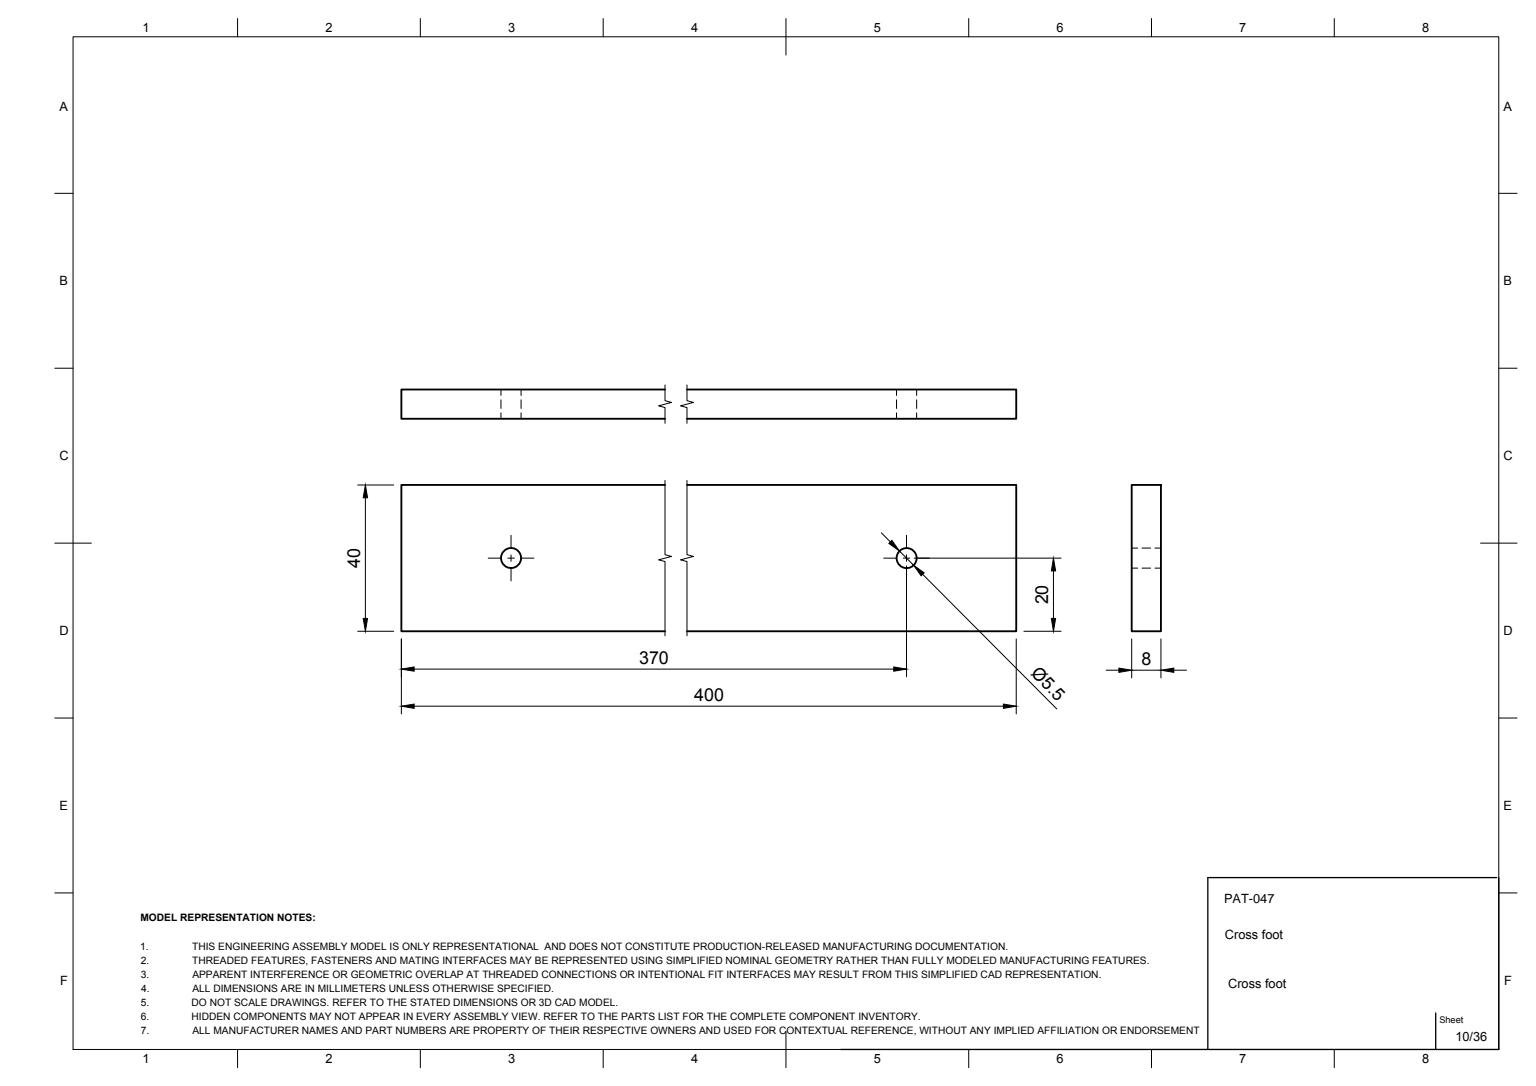
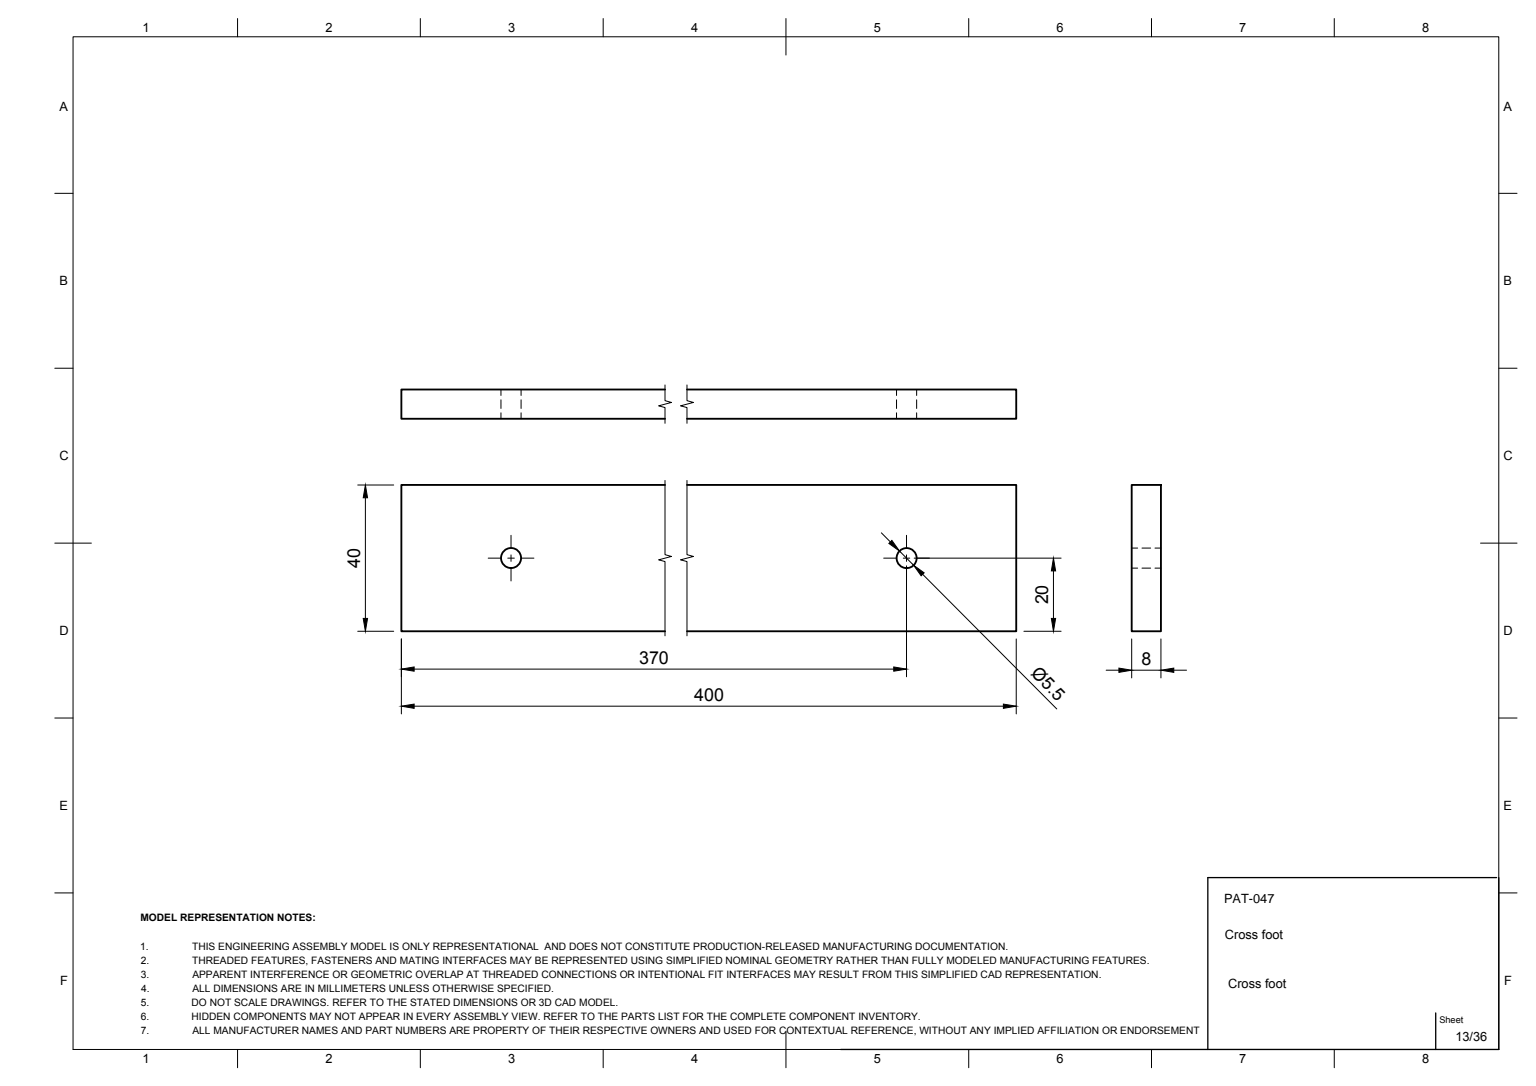
ISO-10303-21;
HEADER;
/* Generated by software containing ST-Developer
 * from STEP Tools, Inc. (www.steptools.com) 
 */

FILE_DESCRIPTION(
/* description */ ('Gravity roller conveyor section'),
/* implementation_level */ '2;1');

FILE_NAME(
/* name */ 'Cross foot.step',
/* time_stamp */ '2026-11-02T07:43:02-08:00',
/* author */ (''),
/* organization */ (''),
/* preprocessor_version */ 'ST-DEVELOPER v20.2',
/* originating_system */ 'Autodesk Translation Framework v15.17.0.0',
/* authorisation */ '');

FILE_SCHEMA (('AUTOMOTIVE_DESIGN { 1 0 10303 214 3 1 1 }'));
ENDSEC;

DATA;
#10=MECHANICAL_DESIGN_GEOMETRIC_PRESENTATION_REPRESENTATION('',(#537),#13821);
#469=SHAPE_REPRESENTATION_RELATIONSHIP('SRR','None',#14006,#503);
#503=ADVANCED_BREP_SHAPE_REPRESENTATION('',(#577),#13793);
#537=STYLED_ITEM('',(#14194),#577);
#577=MANIFOLD_SOLID_BREP('Body1',#7637);
#642=FACE_BOUND('',#1671,.T.);
#643=FACE_BOUND('',#1672,.T.);
#644=FACE_BOUND('',#1674,.T.);
#645=FACE_BOUND('',#1675,.T.);
#877=PLANE('',#8318);
#878=PLANE('',#8319);
#879=PLANE('',#8320);
#880=PLANE('',#8321);
#881=PLANE('',#8322);
#882=PLANE('',#8323);
#1212=FACE_OUTER_BOUND('',#1664,.T.);
#1213=FACE_OUTER_BOUND('',#1665,.T.);
#1214=FACE_OUTER_BOUND('',#1666,.T.);
#1215=FACE_OUTER_BOUND('',#1667,.T.);
#1216=FACE_OUTER_BOUND('',#1668,.T.);
#1217=FACE_OUTER_BOUND('',#1669,.T.);
#1218=FACE_OUTER_BOUND('',#1670,.T.);
#1219=FACE_OUTER_BOUND('',#1673,.T.);
#1664=EDGE_LOOP('',(#6294,#6295,#6296,#6297));
#1665=EDGE_LOOP('',(#6298,#6299,#6300,#6301));
#1666=EDGE_LOOP('',(#6302,#6303,#6304,#6305));
#1667=EDGE_LOOP('',(#6306,#6307,#6308,#6309));
#1668=EDGE_LOOP('',(#6310,#6311,#6312,#6313));
#1669=EDGE_LOOP('',(#6314,#6315,#6316,#6317));
#1670=EDGE_LOOP('',(#6318,#6319,#6320,#6321));
#1671=EDGE_LOOP('',(#6322));
#1672=EDGE_LOOP('',(#6323));
#1673=EDGE_LOOP('',(#6324,#6325,#6326,#6327));
#1674=EDGE_LOOP('',(#6328));
#1675=EDGE_LOOP('',(#6329));
#2426=LINE('',#12371,#3144);
#2427=LINE('',#12377,#3145);
#2428=LINE('',#12382,#3146);
#2429=LINE('',#12384,#3147);
#2430=LINE('',#12386,#3148);
#2431=LINE('',#12387,#3149);
#2432=LINE('',#12390,#3150);
#2433=LINE('',#12392,#3151);
#2434=LINE('',#12393,#3152);
#2435=LINE('',#12396,#3153);
#2436=LINE('',#12398,#3154);
#2437=LINE('',#12399,#3155);
#2438=LINE('',#12401,#3156);
#2439=LINE('',#12402,#3157);
#3144=VECTOR('',#9837,0.275);
#3145=VECTOR('',#9844,0.275);
#3146=VECTOR('',#9849,1.);
#3147=VECTOR('',#9850,1.);
#3148=VECTOR('',#9851,1.);
#3149=VECTOR('',#9852,1.);
#3150=VECTOR('',#9855,1.);
#3151=VECTOR('',#9856,1.);
#3152=VECTOR('',#9857,1.);
#3153=VECTOR('',#9860,1.);
#3154=VECTOR('',#9861,1.);
#3155=VECTOR('',#9862,1.);
#3156=VECTOR('',#9865,1.);
#3157=VECTOR('',#9866,1.);
#3422=CIRCLE('',#8313,0.275);
#3423=CIRCLE('',#8314,0.275);
#3424=CIRCLE('',#8316,0.275);
#3425=CIRCLE('',#8317,0.275);
#3952=VERTEX_POINT('',#12368);
#3953=VERTEX_POINT('',#12370);
#3954=VERTEX_POINT('',#12374);
#3955=VERTEX_POINT('',#12376);
#3956=VERTEX_POINT('',#12380);
#3957=VERTEX_POINT('',#12381);
#3958=VERTEX_POINT('',#12383);
#3959=VERTEX_POINT('',#12385);
#3960=VERTEX_POINT('',#12389);
#3961=VERTEX_POINT('',#12391);
#3962=VERTEX_POINT('',#12395);
#3963=VERTEX_POINT('',#12397);
#4784=EDGE_CURVE('',#3952,#3952,#3422,.T.);
#4785=EDGE_CURVE('',#3952,#3953,#2426,.T.);
#4786=EDGE_CURVE('',#3953,#3953,#3423,.T.);
#4787=EDGE_CURVE('',#3954,#3954,#3424,.T.);
#4788=EDGE_CURVE('',#3954,#3955,#2427,.T.);
#4789=EDGE_CURVE('',#3955,#3955,#3425,.T.);
#4790=EDGE_CURVE('',#3956,#3957,#2428,.T.);
#4791=EDGE_CURVE('',#3957,#3958,#2429,.T.);
#4792=EDGE_CURVE('',#3959,#3958,#2430,.T.);
#4793=EDGE_CURVE('',#3956,#3959,#2431,.T.);
#4794=EDGE_CURVE('',#3960,#3956,#2432,.T.);
#4795=EDGE_CURVE('',#3961,#3959,#2433,.T.);
#4796=EDGE_CURVE('',#3960,#3961,#2434,.T.);
#4797=EDGE_CURVE('',#3962,#3960,#2435,.T.);
#4798=EDGE_CURVE('',#3963,#3961,#2436,.T.);
#4799=EDGE_CURVE('',#3962,#3963,#2437,.T.);
#4800=EDGE_CURVE('',#3957,#3962,#2438,.T.);
#4801=EDGE_CURVE('',#3958,#3963,#2439,.T.);
#6294=ORIENTED_EDGE('',*,*,#4784,.F.);
#6295=ORIENTED_EDGE('',*,*,#4785,.T.);
#6296=ORIENTED_EDGE('',*,*,#4786,.F.);
#6297=ORIENTED_EDGE('',*,*,#4785,.F.);
#6298=ORIENTED_EDGE('',*,*,#4787,.F.);
#6299=ORIENTED_EDGE('',*,*,#4788,.T.);
#6300=ORIENTED_EDGE('',*,*,#4789,.F.);
#6301=ORIENTED_EDGE('',*,*,#4788,.F.);
#6302=ORIENTED_EDGE('',*,*,#4790,.T.);
#6303=ORIENTED_EDGE('',*,*,#4791,.T.);
#6304=ORIENTED_EDGE('',*,*,#4792,.F.);
#6305=ORIENTED_EDGE('',*,*,#4793,.F.);
#6306=ORIENTED_EDGE('',*,*,#4794,.T.);
#6307=ORIENTED_EDGE('',*,*,#4793,.T.);
#6308=ORIENTED_EDGE('',*,*,#4795,.F.);
#6309=ORIENTED_EDGE('',*,*,#4796,.F.);
#6310=ORIENTED_EDGE('',*,*,#4797,.T.);
#6311=ORIENTED_EDGE('',*,*,#4796,.T.);
#6312=ORIENTED_EDGE('',*,*,#4798,.F.);
#6313=ORIENTED_EDGE('',*,*,#4799,.F.);
#6314=ORIENTED_EDGE('',*,*,#4800,.T.);
#6315=ORIENTED_EDGE('',*,*,#4799,.T.);
#6316=ORIENTED_EDGE('',*,*,#4801,.F.);
#6317=ORIENTED_EDGE('',*,*,#4791,.F.);
#6318=ORIENTED_EDGE('',*,*,#4801,.T.);
#6319=ORIENTED_EDGE('',*,*,#4798,.T.);
#6320=ORIENTED_EDGE('',*,*,#4795,.T.);
#6321=ORIENTED_EDGE('',*,*,#4792,.T.);
#6322=ORIENTED_EDGE('',*,*,#4786,.T.);
#6323=ORIENTED_EDGE('',*,*,#4789,.T.);
#6324=ORIENTED_EDGE('',*,*,#4800,.F.);
#6325=ORIENTED_EDGE('',*,*,#4790,.F.);
#6326=ORIENTED_EDGE('',*,*,#4794,.F.);
#6327=ORIENTED_EDGE('',*,*,#4797,.F.);
#6328=ORIENTED_EDGE('',*,*,#4784,.T.);
#6329=ORIENTED_EDGE('',*,*,#4787,.T.);
#7152=CYLINDRICAL_SURFACE('',#8312,0.275);
#7153=CYLINDRICAL_SURFACE('',#8315,0.275);
#7413=ADVANCED_FACE('',(#1212),#7152,.F.);
#7414=ADVANCED_FACE('',(#1213),#7153,.F.);
#7415=ADVANCED_FACE('',(#1214),#877,.T.);
#7416=ADVANCED_FACE('',(#1215),#878,.T.);
#7417=ADVANCED_FACE('',(#1216),#879,.T.);
#7418=ADVANCED_FACE('',(#1217),#880,.T.);
#7419=ADVANCED_FACE('',(#1218,#642,#643),#881,.T.);
#7420=ADVANCED_FACE('',(#1219,#644,#645),#882,.F.);
#7637=CLOSED_SHELL('',(#7413,#7414,#7415,#7416,#7417,#7418,#7419,#7420));
#8311=AXIS2_PLACEMENT_3D('',#12366,#9831,#9832);
#8312=AXIS2_PLACEMENT_3D('',#12367,#9833,#9834);
#8313=AXIS2_PLACEMENT_3D('',#12369,#9835,#9836);
#8314=AXIS2_PLACEMENT_3D('',#12372,#9838,#9839);
#8315=AXIS2_PLACEMENT_3D('',#12373,#9840,#9841);
#8316=AXIS2_PLACEMENT_3D('',#12375,#9842,#9843);
#8317=AXIS2_PLACEMENT_3D('',#12378,#9845,#9846);
#8318=AXIS2_PLACEMENT_3D('',#12379,#9847,#9848);
#8319=AXIS2_PLACEMENT_3D('',#12388,#9853,#9854);
#8320=AXIS2_PLACEMENT_3D('',#12394,#9858,#9859);
#8321=AXIS2_PLACEMENT_3D('',#12400,#9863,#9864);
#8322=AXIS2_PLACEMENT_3D('',#12403,#9867,#9868);
#8323=AXIS2_PLACEMENT_3D('',#12404,#9869,#9870);
#9831=DIRECTION('axis',(0.,0.,1.));
#9832=DIRECTION('refdir',(1.,0.,0.));
#9833=DIRECTION('center_axis',(0.,0.,1.));
#9834=DIRECTION('ref_axis',(1.,0.,0.));
#9835=DIRECTION('center_axis',(0.,0.,1.));
#9836=DIRECTION('ref_axis',(1.,0.,0.));
#9837=DIRECTION('',(0.,0.,1.));
#9838=DIRECTION('center_axis',(0.,0.,-1.));
#9839=DIRECTION('ref_axis',(1.,0.,0.));
#9840=DIRECTION('center_axis',(0.,0.,1.));
#9841=DIRECTION('ref_axis',(1.,0.,0.));
#9842=DIRECTION('center_axis',(0.,0.,1.));
#9843=DIRECTION('ref_axis',(1.,0.,0.));
#9844=DIRECTION('',(0.,0.,1.));
#9845=DIRECTION('center_axis',(0.,0.,-1.));
#9846=DIRECTION('ref_axis',(1.,0.,0.));
#9847=DIRECTION('center_axis',(0.,1.,0.));
#9848=DIRECTION('ref_axis',(-1.,0.,0.));
#9849=DIRECTION('',(-1.,0.,0.));
#9850=DIRECTION('',(0.,0.,1.));
#9851=DIRECTION('',(-1.,0.,0.));
#9852=DIRECTION('',(0.,0.,1.));
#9853=DIRECTION('center_axis',(1.,0.,0.));
#9854=DIRECTION('ref_axis',(0.,1.,0.));
#9855=DIRECTION('',(0.,1.,0.));
#9856=DIRECTION('',(0.,1.,0.));
#9857=DIRECTION('',(0.,0.,1.));
#9858=DIRECTION('center_axis',(0.,-1.,0.));
#9859=DIRECTION('ref_axis',(1.,0.,0.));
#9860=DIRECTION('',(1.,0.,0.));
#9861=DIRECTION('',(1.,0.,0.));
#9862=DIRECTION('',(0.,0.,1.));
#9863=DIRECTION('center_axis',(-1.,0.,0.));
#9864=DIRECTION('ref_axis',(0.,-1.,0.));
#9865=DIRECTION('',(0.,-1.,0.));
#9866=DIRECTION('',(0.,-1.,0.));
#9867=DIRECTION('center_axis',(0.,0.,1.));
#9868=DIRECTION('ref_axis',(1.,0.,0.));
#9869=DIRECTION('center_axis',(0.,0.,1.));
#9870=DIRECTION('ref_axis',(1.,0.,0.));
#12366=CARTESIAN_POINT('',(0.,0.,0.));
#12367=CARTESIAN_POINT('Origin',(6.,-2.,-16.9));
#12368=CARTESIAN_POINT('',(5.725,-2.,-16.8));
#12369=CARTESIAN_POINT('Origin',(6.,-2.,-16.8));
#12370=CARTESIAN_POINT('',(5.725,-2.,-16.));
#12371=CARTESIAN_POINT('',(5.725,-2.,-16.9));
#12372=CARTESIAN_POINT('Origin',(6.,-2.,-16.));
#12373=CARTESIAN_POINT('Origin',(6.,32.,-16.9));
#12374=CARTESIAN_POINT('',(5.725,32.,-16.8));
#12375=CARTESIAN_POINT('Origin',(6.,32.,-16.8));
#12376=CARTESIAN_POINT('',(5.725,32.,-16.));
#12377=CARTESIAN_POINT('',(5.725,32.,-16.9));
#12378=CARTESIAN_POINT('Origin',(6.,32.,-16.));
#12379=CARTESIAN_POINT('Origin',(8.,35.,-16.8));
#12380=CARTESIAN_POINT('',(8.,35.,-16.8));
#12381=CARTESIAN_POINT('',(4.,35.,-16.8));
#12382=CARTESIAN_POINT('',(8.,35.,-16.8));
#12383=CARTESIAN_POINT('',(4.,35.,-16.));
#12384=CARTESIAN_POINT('',(4.,35.,-16.8));
#12385=CARTESIAN_POINT('',(8.,35.,-16.));
#12386=CARTESIAN_POINT('',(8.,35.,-16.));
#12387=CARTESIAN_POINT('',(8.,35.,-16.8));
#12388=CARTESIAN_POINT('Origin',(8.,-5.,-16.8));
#12389=CARTESIAN_POINT('',(8.,-5.,-16.8));
#12390=CARTESIAN_POINT('',(8.,-5.,-16.8));
#12391=CARTESIAN_POINT('',(8.,-5.,-16.));
#12392=CARTESIAN_POINT('',(8.,-5.,-16.));
#12393=CARTESIAN_POINT('',(8.,-5.,-16.8));
#12394=CARTESIAN_POINT('Origin',(4.,-5.,-16.8));
#12395=CARTESIAN_POINT('',(4.,-5.,-16.8));
#12396=CARTESIAN_POINT('',(4.,-5.,-16.8));
#12397=CARTESIAN_POINT('',(4.,-5.,-16.));
#12398=CARTESIAN_POINT('',(4.,-5.,-16.));
#12399=CARTESIAN_POINT('',(4.,-5.,-16.8));
#12400=CARTESIAN_POINT('Origin',(4.,35.,-16.8));
#12401=CARTESIAN_POINT('',(4.,35.,-16.8));
#12402=CARTESIAN_POINT('',(4.,35.,-16.));
#12403=CARTESIAN_POINT('Origin',(6.,15.,-16.));
#12404=CARTESIAN_POINT('Origin',(6.,15.,-16.8));
#13754=UNCERTAINTY_MEASURE_WITH_UNIT(LENGTH_MEASURE(0.001),#13822,
'DISTANCE_ACCURACY_VALUE',
'Maximum model space distance between geometric entities at asserted c
onnectivities');
#13782=UNCERTAINTY_MEASURE_WITH_UNIT(LENGTH_MEASURE(0.001),#13822,
'DISTANCE_ACCURACY_VALUE',
'Maximum model space distance between geometric entities at asserted c
onnectivities');
#13793=(
GEOMETRIC_REPRESENTATION_CONTEXT(3)
GLOBAL_UNCERTAINTY_ASSIGNED_CONTEXT((#13754))
GLOBAL_UNIT_ASSIGNED_CONTEXT((#13822,#13824,#13825))
REPRESENTATION_CONTEXT('','3D')
);
#13821=(
GEOMETRIC_REPRESENTATION_CONTEXT(3)
GLOBAL_UNCERTAINTY_ASSIGNED_CONTEXT((#13782))
GLOBAL_UNIT_ASSIGNED_CONTEXT((#13822,#13824,#13825))
REPRESENTATION_CONTEXT('','3D')
);
#13822=(
LENGTH_UNIT()
NAMED_UNIT(*)
SI_UNIT(.CENTI.,.METRE.)
);
#13824=(
NAMED_UNIT(*)
PLANE_ANGLE_UNIT()
SI_UNIT($,.RADIAN.)
);
#13825=(
NAMED_UNIT(*)
SI_UNIT($,.STERADIAN.)
SOLID_ANGLE_UNIT()
);
#13836=SHAPE_DEFINITION_REPRESENTATION(#13874,#14006);
#13874=PRODUCT_DEFINITION_SHAPE('',$,#14045);
#14006=SHAPE_REPRESENTATION('',(#8311),#13793);
#14034=PRODUCT_DEFINITION_CONTEXT('part definition',#14150,'design');
#14045=PRODUCT_DEFINITION('Cross foot','Cross foot',#14083,#14034);
#14083=PRODUCT_DEFINITION_FORMATION('',$,#14162);
#14150=APPLICATION_CONTEXT(
'Core Data for Automotive Mechanical Design Process');
#14151=PRODUCT_CONTEXT('part definition',#14150,'mechanical');
#14162=PRODUCT('Cross foot','Cross foot','Cross foot',(#14151));
#14194=PRESENTATION_STYLE_ASSIGNMENT((#14199));
#14199=SURFACE_STYLE_USAGE(.BOTH.,#14204);
#14204=SURFACE_SIDE_STYLE('',(#14209));
#14209=SURFACE_STYLE_FILL_AREA(#14214);
#14214=FILL_AREA_STYLE('CAD Library Painted - Deep blue',(#14219));
#14219=FILL_AREA_STYLE_COLOUR('CAD Library Painted - Deep blue',#14224);
#14224=COLOUR_RGB('CAD Library Painted - Deep blue',0.0784313725490196,
0.203921568627451,0.349019607843137);
ENDSEC;
END-ISO-10303-21;
